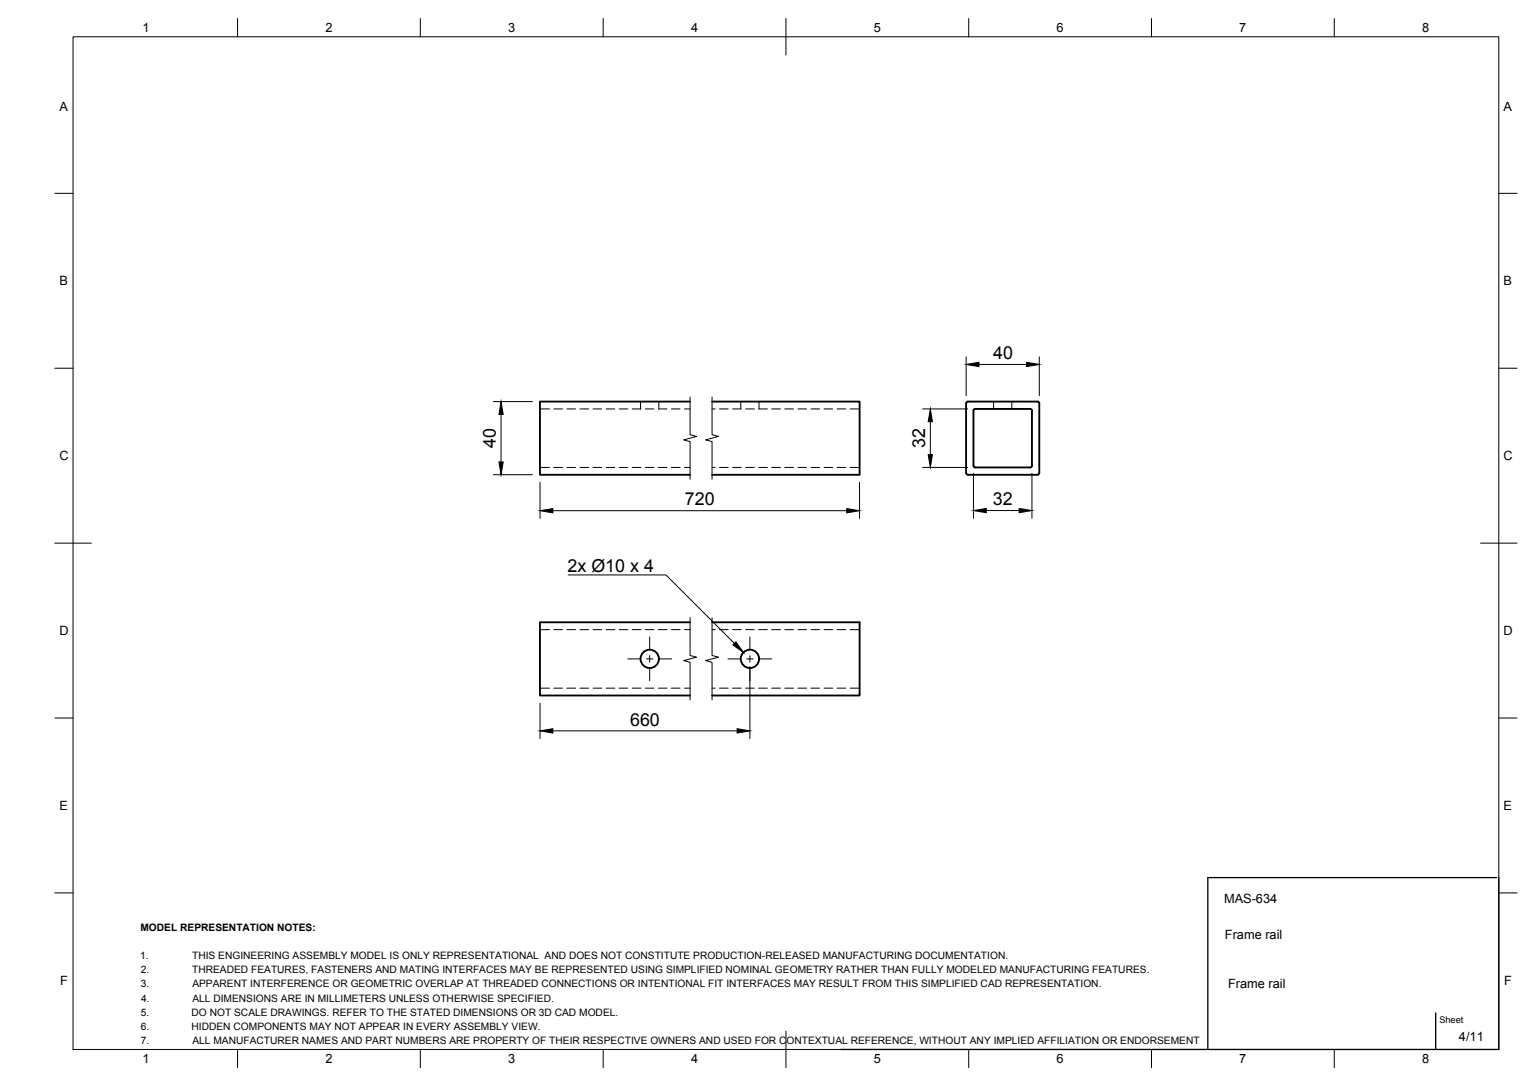
ISO-10303-21;
HEADER;
/* Generated by software containing ST-Developer
 * from STEP Tools, Inc. (www.steptools.com) 
 */

FILE_DESCRIPTION(
/* description */ ('Independent AHU equipment rack. Nominal800x600 frame on1000long40squa
re aluminum posts; two removable notched shelves; welded perimeter/cro
ss rails and rear gussets; two mounting channels; four isolation pads 
and anchor-ready feet. Imported native extrusion library retained and 
cut-length parameters customized per family. Shelf hardware uses model
ed M6 rivet nuts and screws. Weld design, floor anchors and load ratin
g require engineering selection.'),
/* implementation_level */ '2;1');

FILE_NAME(
/* name */ 'Frame rail.step',
/* time_stamp */ '2026-11-07T19:04:45-08:00',
/* author */ (''),
/* organization */ (''),
/* preprocessor_version */ 'ST-DEVELOPER v20.2',
/* originating_system */ 'Autodesk Translation Framework v15.17.0.0',
/* authorisation */ '');

FILE_SCHEMA (('AUTOMOTIVE_DESIGN { 1 0 10303 214 3 1 1 }'));
ENDSEC;

DATA;
#10=MECHANICAL_DESIGN_GEOMETRIC_PRESENTATION_REPRESENTATION('',(#336),#9777);
#314=SHAPE_REPRESENTATION_RELATIONSHIP('SRR','None',#9858,#325);
#325=ADVANCED_BREP_SHAPE_REPRESENTATION('',(#347),#9767);
#336=STYLED_ITEM('',(#9922),#347);
#347=MANIFOLD_SOLID_BREP('Aluminum square hollow profile',#3841);
#359=FACE_BOUND('',#725,.T.);
#360=FACE_BOUND('',#732,.T.);
#361=FACE_BOUND('',#733,.T.);
#362=FACE_BOUND('',#741,.T.);
#363=FACE_BOUND('',#742,.T.);
#364=FACE_BOUND('',#745,.T.);
#420=PLANE('',#4019);
#421=PLANE('',#4020);
#422=PLANE('',#4030);
#423=PLANE('',#4037);
#424=PLANE('',#4040);
#425=PLANE('',#4043);
#426=PLANE('',#4046);
#427=PLANE('',#4047);
#428=PLANE('',#4048);
#429=PLANE('',#4049);
#520=FACE_OUTER_BOUND('',#720,.T.);
#521=FACE_OUTER_BOUND('',#721,.T.);
#522=FACE_OUTER_BOUND('',#722,.T.);
#523=FACE_OUTER_BOUND('',#723,.T.);
#524=FACE_OUTER_BOUND('',#724,.T.);
#525=FACE_OUTER_BOUND('',#726,.T.);
#526=FACE_OUTER_BOUND('',#727,.T.);
#527=FACE_OUTER_BOUND('',#728,.T.);
#528=FACE_OUTER_BOUND('',#729,.T.);
#529=FACE_OUTER_BOUND('',#730,.T.);
#530=FACE_OUTER_BOUND('',#731,.T.);
#531=FACE_OUTER_BOUND('',#734,.T.);
#532=FACE_OUTER_BOUND('',#735,.T.);
#533=FACE_OUTER_BOUND('',#736,.T.);
#534=FACE_OUTER_BOUND('',#737,.T.);
#535=FACE_OUTER_BOUND('',#738,.T.);
#536=FACE_OUTER_BOUND('',#739,.T.);
#537=FACE_OUTER_BOUND('',#740,.T.);
#538=FACE_OUTER_BOUND('',#743,.T.);
#539=FACE_OUTER_BOUND('',#744,.T.);
#720=EDGE_LOOP('',(#2611,#2612,#2613,#2614));
#721=EDGE_LOOP('',(#2615,#2616,#2617,#2618));
#722=EDGE_LOOP('',(#2619,#2620,#2621,#2622));
#723=EDGE_LOOP('',(#2623,#2624,#2625,#2626));
#724=EDGE_LOOP('',(#2627,#2628,#2629,#2630,#2631,#2632,#2633,#2634));
#725=EDGE_LOOP('',(#2635,#2636,#2637,#2638,#2639,#2640,#2641,#2642));
#726=EDGE_LOOP('',(#2643,#2644,#2645,#2646));
#727=EDGE_LOOP('',(#2647,#2648,#2649,#2650));
#728=EDGE_LOOP('',(#2651,#2652,#2653,#2654));
#729=EDGE_LOOP('',(#2655,#2656,#2657,#2658));
#730=EDGE_LOOP('',(#2659,#2660,#2661,#2662));
#731=EDGE_LOOP('',(#2663,#2664,#2665,#2666));
#732=EDGE_LOOP('',(#2667));
#733=EDGE_LOOP('',(#2668));
#734=EDGE_LOOP('',(#2669,#2670,#2671,#2672));
#735=EDGE_LOOP('',(#2673,#2674,#2675,#2676));
#736=EDGE_LOOP('',(#2677,#2678,#2679,#2680));
#737=EDGE_LOOP('',(#2681,#2682,#2683,#2684));
#738=EDGE_LOOP('',(#2685,#2686,#2687,#2688));
#739=EDGE_LOOP('',(#2689,#2690,#2691,#2692));
#740=EDGE_LOOP('',(#2693,#2694,#2695,#2696));
#741=EDGE_LOOP('',(#2697));
#742=EDGE_LOOP('',(#2698));
#743=EDGE_LOOP('',(#2699,#2700,#2701,#2702));
#744=EDGE_LOOP('',(#2703,#2704,#2705,#2706,#2707,#2708,#2709,#2710));
#745=EDGE_LOOP('',(#2711,#2712,#2713,#2714,#2715,#2716,#2717,#2718));
#983=LINE('',#5508,#1276);
#984=LINE('',#5514,#1277);
#985=LINE('',#5521,#1278);
#986=LINE('',#5524,#1279);
#987=LINE('',#5527,#1280);
#988=LINE('',#5529,#1281);
#989=LINE('',#5530,#1282);
#990=LINE('',#5533,#1283);
#991=LINE('',#5537,#1284);
#992=LINE('',#5541,#1285);
#993=LINE('',#5545,#1286);
#994=LINE('',#5549,#1287);
#995=LINE('',#5553,#1288);
#996=LINE('',#5557,#1289);
#997=LINE('',#5561,#1290);
#998=LINE('',#5564,#1291);
#999=LINE('',#5567,#1292);
#1000=LINE('',#5568,#1293);
#1001=LINE('',#5572,#1294);
#1002=LINE('',#5575,#1295);
#1003=LINE('',#5581,#1296);
#1004=LINE('',#5582,#1297);
#1005=LINE('',#5585,#1298);
#1006=LINE('',#5586,#1299);
#1007=LINE('',#5590,#1300);
#1008=LINE('',#5593,#1301);
#1009=LINE('',#5594,#1302);
#1010=LINE('',#5598,#1303);
#1011=LINE('',#5601,#1304);
#1012=LINE('',#5602,#1305);
#1013=LINE('',#5606,#1306);
#1014=LINE('',#5608,#1307);
#1015=LINE('',#5610,#1308);
#1016=LINE('',#5612,#1309);
#1276=VECTOR('',#4462,5.);
#1277=VECTOR('',#4469,5.);
#1278=VECTOR('',#4476,10.);
#1279=VECTOR('',#4479,10.);
#1280=VECTOR('',#4482,10.);
#1281=VECTOR('',#4483,10.);
#1282=VECTOR('',#4484,10.);
#1283=VECTOR('',#4487,10.);
#1284=VECTOR('',#4490,10.);
#1285=VECTOR('',#4493,10.);
#1286=VECTOR('',#4496,10.);
#1287=VECTOR('',#4499,10.);
#1288=VECTOR('',#4502,10.);
#1289=VECTOR('',#4505,10.);
#1290=VECTOR('',#4510,10.);
#1291=VECTOR('',#4513,10.);
#1292=VECTOR('',#4516,10.);
#1293=VECTOR('',#4517,10.);
#1294=VECTOR('',#4522,10.);
#1295=VECTOR('',#4525,10.);
#1296=VECTOR('',#4532,10.);
#1297=VECTOR('',#4533,10.);
#1298=VECTOR('',#4536,10.);
#1299=VECTOR('',#4537,10.);
#1300=VECTOR('',#4542,10.);
#1301=VECTOR('',#4545,10.);
#1302=VECTOR('',#4546,10.);
#1303=VECTOR('',#4551,10.);
#1304=VECTOR('',#4554,10.);
#1305=VECTOR('',#4555,10.);
#1306=VECTOR('',#4560,10.);
#1307=VECTOR('',#4563,10.);
#1308=VECTOR('',#4566,10.);
#1309=VECTOR('',#4569,10.);
#1553=CIRCLE('',#4011,5.);
#1554=CIRCLE('',#4012,5.);
#1555=CIRCLE('',#4014,5.);
#1556=CIRCLE('',#4015,5.);
#1557=CIRCLE('',#4017,1.);
#1558=CIRCLE('',#4018,1.);
#1559=CIRCLE('',#4021,1.);
#1560=CIRCLE('',#4022,1.);
#1561=CIRCLE('',#4023,1.);
#1562=CIRCLE('',#4024,1.);
#1563=CIRCLE('',#4025,1.);
#1564=CIRCLE('',#4026,1.);
#1565=CIRCLE('',#4027,1.);
#1566=CIRCLE('',#4029,1.);
#1567=CIRCLE('',#4032,1.);
#1568=CIRCLE('',#4034,1.);
#1569=CIRCLE('',#4036,1.);
#1570=CIRCLE('',#4039,1.);
#1571=CIRCLE('',#4042,1.);
#1572=CIRCLE('',#4045,1.);
#1692=VERTEX_POINT('',#5505);
#1693=VERTEX_POINT('',#5507);
#1694=VERTEX_POINT('',#5511);
#1695=VERTEX_POINT('',#5513);
#1696=VERTEX_POINT('',#5517);
#1697=VERTEX_POINT('',#5518);
#1698=VERTEX_POINT('',#5520);
#1699=VERTEX_POINT('',#5522);
#1700=VERTEX_POINT('',#5526);
#1701=VERTEX_POINT('',#5528);
#1702=VERTEX_POINT('',#5532);
#1703=VERTEX_POINT('',#5534);
#1704=VERTEX_POINT('',#5536);
#1705=VERTEX_POINT('',#5538);
#1706=VERTEX_POINT('',#5540);
#1707=VERTEX_POINT('',#5543);
#1708=VERTEX_POINT('',#5544);
#1709=VERTEX_POINT('',#5546);
#1710=VERTEX_POINT('',#5548);
#1711=VERTEX_POINT('',#5550);
#1712=VERTEX_POINT('',#5552);
#1713=VERTEX_POINT('',#5554);
#1714=VERTEX_POINT('',#5556);
#1715=VERTEX_POINT('',#5560);
#1716=VERTEX_POINT('',#5562);
#1717=VERTEX_POINT('',#5566);
#1718=VERTEX_POINT('',#5570);
#1719=VERTEX_POINT('',#5574);
#1720=VERTEX_POINT('',#5578);
#1721=VERTEX_POINT('',#5579);
#1722=VERTEX_POINT('',#5584);
#1723=VERTEX_POINT('',#5588);
#1724=VERTEX_POINT('',#5592);
#1725=VERTEX_POINT('',#5596);
#1726=VERTEX_POINT('',#5600);
#1727=VERTEX_POINT('',#5604);
#2050=EDGE_CURVE('',#1692,#1692,#1553,.T.);
#2051=EDGE_CURVE('',#1692,#1693,#983,.T.);
#2052=EDGE_CURVE('',#1693,#1693,#1554,.T.);
#2053=EDGE_CURVE('',#1694,#1694,#1555,.T.);
#2054=EDGE_CURVE('',#1694,#1695,#984,.T.);
#2055=EDGE_CURVE('',#1695,#1695,#1556,.T.);
#2056=EDGE_CURVE('',#1696,#1697,#1557,.T.);
#2057=EDGE_CURVE('',#1697,#1698,#985,.T.);
#2058=EDGE_CURVE('',#1698,#1699,#1558,.T.);
#2059=EDGE_CURVE('',#1699,#1696,#986,.T.);
#2060=EDGE_CURVE('',#1700,#1697,#987,.T.);
#2061=EDGE_CURVE('',#1701,#1700,#988,.T.);
#2062=EDGE_CURVE('',#1701,#1698,#989,.T.);
#2063=EDGE_CURVE('',#1696,#1702,#990,.T.);
#2064=EDGE_CURVE('',#1703,#1702,#1559,.T.);
#2065=EDGE_CURVE('',#1703,#1704,#991,.T.);
#2066=EDGE_CURVE('',#1705,#1704,#1560,.T.);
#2067=EDGE_CURVE('',#1705,#1706,#992,.T.);
#2068=EDGE_CURVE('',#1700,#1706,#1561,.T.);
#2069=EDGE_CURVE('',#1707,#1708,#993,.T.);
#2070=EDGE_CURVE('',#1709,#1708,#1562,.T.);
#2071=EDGE_CURVE('',#1709,#1710,#994,.T.);
#2072=EDGE_CURVE('',#1711,#1710,#1563,.T.);
#2073=EDGE_CURVE('',#1711,#1712,#995,.T.);
#2074=EDGE_CURVE('',#1713,#1712,#1564,.T.);
#2075=EDGE_CURVE('',#1713,#1714,#996,.T.);
#2076=EDGE_CURVE('',#1707,#1714,#1565,.T.);
#2077=EDGE_CURVE('',#1702,#1715,#997,.T.);
#2078=EDGE_CURVE('',#1715,#1716,#1566,.T.);
#2079=EDGE_CURVE('',#1716,#1703,#998,.T.);
#2080=EDGE_CURVE('',#1716,#1717,#999,.T.);
#2081=EDGE_CURVE('',#1704,#1717,#1000,.T.);
#2082=EDGE_CURVE('',#1717,#1718,#1567,.T.);
#2083=EDGE_CURVE('',#1718,#1705,#1001,.T.);
#2084=EDGE_CURVE('',#1706,#1719,#1002,.T.);
#2085=EDGE_CURVE('',#1719,#1701,#1568,.T.);
#2086=EDGE_CURVE('',#1720,#1721,#1569,.T.);
#2087=EDGE_CURVE('',#1721,#1709,#1003,.T.);
#2088=EDGE_CURVE('',#1708,#1720,#1004,.T.);
#2089=EDGE_CURVE('',#1721,#1722,#1005,.T.);
#2090=EDGE_CURVE('',#1710,#1722,#1006,.T.);
#2091=EDGE_CURVE('',#1722,#1723,#1570,.T.);
#2092=EDGE_CURVE('',#1723,#1711,#1007,.T.);
#2093=EDGE_CURVE('',#1723,#1724,#1008,.T.);
#2094=EDGE_CURVE('',#1712,#1724,#1009,.T.);
#2095=EDGE_CURVE('',#1724,#1725,#1571,.T.);
#2096=EDGE_CURVE('',#1725,#1713,#1010,.T.);
#2097=EDGE_CURVE('',#1725,#1726,#1011,.T.);
#2098=EDGE_CURVE('',#1714,#1726,#1012,.T.);
#2099=EDGE_CURVE('',#1726,#1727,#1572,.T.);
#2100=EDGE_CURVE('',#1727,#1707,#1013,.T.);
#2101=EDGE_CURVE('',#1727,#1720,#1014,.T.);
#2102=EDGE_CURVE('',#1718,#1719,#1015,.T.);
#2103=EDGE_CURVE('',#1699,#1715,#1016,.T.);
#2611=ORIENTED_EDGE('',*,*,#2050,.F.);
#2612=ORIENTED_EDGE('',*,*,#2051,.T.);
#2613=ORIENTED_EDGE('',*,*,#2052,.F.);
#2614=ORIENTED_EDGE('',*,*,#2051,.F.);
#2615=ORIENTED_EDGE('',*,*,#2053,.F.);
#2616=ORIENTED_EDGE('',*,*,#2054,.T.);
#2617=ORIENTED_EDGE('',*,*,#2055,.F.);
#2618=ORIENTED_EDGE('',*,*,#2054,.F.);
#2619=ORIENTED_EDGE('',*,*,#2056,.T.);
#2620=ORIENTED_EDGE('',*,*,#2057,.T.);
#2621=ORIENTED_EDGE('',*,*,#2058,.T.);
#2622=ORIENTED_EDGE('',*,*,#2059,.T.);
#2623=ORIENTED_EDGE('',*,*,#2057,.F.);
#2624=ORIENTED_EDGE('',*,*,#2060,.F.);
#2625=ORIENTED_EDGE('',*,*,#2061,.F.);
#2626=ORIENTED_EDGE('',*,*,#2062,.T.);
#2627=ORIENTED_EDGE('',*,*,#2056,.F.);
#2628=ORIENTED_EDGE('',*,*,#2063,.T.);
#2629=ORIENTED_EDGE('',*,*,#2064,.F.);
#2630=ORIENTED_EDGE('',*,*,#2065,.T.);
#2631=ORIENTED_EDGE('',*,*,#2066,.F.);
#2632=ORIENTED_EDGE('',*,*,#2067,.T.);
#2633=ORIENTED_EDGE('',*,*,#2068,.F.);
#2634=ORIENTED_EDGE('',*,*,#2060,.T.);
#2635=ORIENTED_EDGE('',*,*,#2069,.T.);
#2636=ORIENTED_EDGE('',*,*,#2070,.F.);
#2637=ORIENTED_EDGE('',*,*,#2071,.T.);
#2638=ORIENTED_EDGE('',*,*,#2072,.F.);
#2639=ORIENTED_EDGE('',*,*,#2073,.T.);
#2640=ORIENTED_EDGE('',*,*,#2074,.F.);
#2641=ORIENTED_EDGE('',*,*,#2075,.T.);
#2642=ORIENTED_EDGE('',*,*,#2076,.F.);
#2643=ORIENTED_EDGE('',*,*,#2064,.T.);
#2644=ORIENTED_EDGE('',*,*,#2077,.T.);
#2645=ORIENTED_EDGE('',*,*,#2078,.T.);
#2646=ORIENTED_EDGE('',*,*,#2079,.T.);
#2647=ORIENTED_EDGE('',*,*,#2079,.F.);
#2648=ORIENTED_EDGE('',*,*,#2080,.T.);
#2649=ORIENTED_EDGE('',*,*,#2081,.F.);
#2650=ORIENTED_EDGE('',*,*,#2065,.F.);
#2651=ORIENTED_EDGE('',*,*,#2066,.T.);
#2652=ORIENTED_EDGE('',*,*,#2081,.T.);
#2653=ORIENTED_EDGE('',*,*,#2082,.T.);
#2654=ORIENTED_EDGE('',*,*,#2083,.T.);
#2655=ORIENTED_EDGE('',*,*,#2068,.T.);
#2656=ORIENTED_EDGE('',*,*,#2084,.T.);
#2657=ORIENTED_EDGE('',*,*,#2085,.T.);
#2658=ORIENTED_EDGE('',*,*,#2061,.T.);
#2659=ORIENTED_EDGE('',*,*,#2086,.T.);
#2660=ORIENTED_EDGE('',*,*,#2087,.T.);
#2661=ORIENTED_EDGE('',*,*,#2070,.T.);
#2662=ORIENTED_EDGE('',*,*,#2088,.T.);
#2663=ORIENTED_EDGE('',*,*,#2087,.F.);
#2664=ORIENTED_EDGE('',*,*,#2089,.T.);
#2665=ORIENTED_EDGE('',*,*,#2090,.F.);
#2666=ORIENTED_EDGE('',*,*,#2071,.F.);
#2667=ORIENTED_EDGE('',*,*,#2052,.T.);
#2668=ORIENTED_EDGE('',*,*,#2055,.T.);
#2669=ORIENTED_EDGE('',*,*,#2091,.T.);
#2670=ORIENTED_EDGE('',*,*,#2092,.T.);
#2671=ORIENTED_EDGE('',*,*,#2072,.T.);
#2672=ORIENTED_EDGE('',*,*,#2090,.T.);
#2673=ORIENTED_EDGE('',*,*,#2092,.F.);
#2674=ORIENTED_EDGE('',*,*,#2093,.T.);
#2675=ORIENTED_EDGE('',*,*,#2094,.F.);
#2676=ORIENTED_EDGE('',*,*,#2073,.F.);
#2677=ORIENTED_EDGE('',*,*,#2095,.T.);
#2678=ORIENTED_EDGE('',*,*,#2096,.T.);
#2679=ORIENTED_EDGE('',*,*,#2074,.T.);
#2680=ORIENTED_EDGE('',*,*,#2094,.T.);
#2681=ORIENTED_EDGE('',*,*,#2096,.F.);
#2682=ORIENTED_EDGE('',*,*,#2097,.T.);
#2683=ORIENTED_EDGE('',*,*,#2098,.F.);
#2684=ORIENTED_EDGE('',*,*,#2075,.F.);
#2685=ORIENTED_EDGE('',*,*,#2099,.T.);
#2686=ORIENTED_EDGE('',*,*,#2100,.T.);
#2687=ORIENTED_EDGE('',*,*,#2076,.T.);
#2688=ORIENTED_EDGE('',*,*,#2098,.T.);
#2689=ORIENTED_EDGE('',*,*,#2088,.F.);
#2690=ORIENTED_EDGE('',*,*,#2069,.F.);
#2691=ORIENTED_EDGE('',*,*,#2100,.F.);
#2692=ORIENTED_EDGE('',*,*,#2101,.T.);
#2693=ORIENTED_EDGE('',*,*,#2083,.F.);
#2694=ORIENTED_EDGE('',*,*,#2102,.T.);
#2695=ORIENTED_EDGE('',*,*,#2084,.F.);
#2696=ORIENTED_EDGE('',*,*,#2067,.F.);
#2697=ORIENTED_EDGE('',*,*,#2050,.T.);
#2698=ORIENTED_EDGE('',*,*,#2053,.T.);
#2699=ORIENTED_EDGE('',*,*,#2059,.F.);
#2700=ORIENTED_EDGE('',*,*,#2103,.T.);
#2701=ORIENTED_EDGE('',*,*,#2077,.F.);
#2702=ORIENTED_EDGE('',*,*,#2063,.F.);
#2703=ORIENTED_EDGE('',*,*,#2058,.F.);
#2704=ORIENTED_EDGE('',*,*,#2062,.F.);
#2705=ORIENTED_EDGE('',*,*,#2085,.F.);
#2706=ORIENTED_EDGE('',*,*,#2102,.F.);
#2707=ORIENTED_EDGE('',*,*,#2082,.F.);
#2708=ORIENTED_EDGE('',*,*,#2080,.F.);
#2709=ORIENTED_EDGE('',*,*,#2078,.F.);
#2710=ORIENTED_EDGE('',*,*,#2103,.F.);
#2711=ORIENTED_EDGE('',*,*,#2099,.F.);
#2712=ORIENTED_EDGE('',*,*,#2097,.F.);
#2713=ORIENTED_EDGE('',*,*,#2095,.F.);
#2714=ORIENTED_EDGE('',*,*,#2093,.F.);
#2715=ORIENTED_EDGE('',*,*,#2091,.F.);
#2716=ORIENTED_EDGE('',*,*,#2089,.F.);
#2717=ORIENTED_EDGE('',*,*,#2086,.F.);
#2718=ORIENTED_EDGE('',*,*,#2101,.F.);
#3549=CYLINDRICAL_SURFACE('',#4010,5.);
#3550=CYLINDRICAL_SURFACE('',#4013,5.);
#3551=CYLINDRICAL_SURFACE('',#4016,1.);
#3552=CYLINDRICAL_SURFACE('',#4028,1.);
#3553=CYLINDRICAL_SURFACE('',#4031,1.);
#3554=CYLINDRICAL_SURFACE('',#4033,1.);
#3555=CYLINDRICAL_SURFACE('',#4035,1.);
#3556=CYLINDRICAL_SURFACE('',#4038,1.);
#3557=CYLINDRICAL_SURFACE('',#4041,1.);
#3558=CYLINDRICAL_SURFACE('',#4044,1.);
#3660=ADVANCED_FACE('',(#520),#3549,.F.);
#3661=ADVANCED_FACE('',(#521),#3550,.F.);
#3662=ADVANCED_FACE('',(#522),#3551,.T.);
#3663=ADVANCED_FACE('',(#523),#420,.T.);
#3664=ADVANCED_FACE('',(#524,#359),#421,.T.);
#3665=ADVANCED_FACE('',(#525),#3552,.T.);
#3666=ADVANCED_FACE('',(#526),#422,.T.);
#3667=ADVANCED_FACE('',(#527),#3553,.T.);
#3668=ADVANCED_FACE('',(#528),#3554,.T.);
#3669=ADVANCED_FACE('',(#529),#3555,.F.);
#3670=ADVANCED_FACE('',(#530,#360,#361),#423,.T.);
#3671=ADVANCED_FACE('',(#531),#3556,.F.);
#3672=ADVANCED_FACE('',(#532),#424,.T.);
#3673=ADVANCED_FACE('',(#533),#3557,.F.);
#3674=ADVANCED_FACE('',(#534),#425,.T.);
#3675=ADVANCED_FACE('',(#535),#3558,.F.);
#3676=ADVANCED_FACE('',(#536),#426,.T.);
#3677=ADVANCED_FACE('',(#537,#362,#363),#427,.T.);
#3678=ADVANCED_FACE('',(#538),#428,.T.);
#3679=ADVANCED_FACE('',(#539,#364),#429,.F.);
#3841=CLOSED_SHELL('',(#3660,#3661,#3662,#3663,#3664,#3665,#3666,#3667,
#3668,#3669,#3670,#3671,#3672,#3673,#3674,#3675,#3676,#3677,#3678,#3679));
#4009=AXIS2_PLACEMENT_3D('',#5503,#4456,#4457);
#4010=AXIS2_PLACEMENT_3D('',#5504,#4458,#4459);
#4011=AXIS2_PLACEMENT_3D('',#5506,#4460,#4461);
#4012=AXIS2_PLACEMENT_3D('',#5509,#4463,#4464);
#4013=AXIS2_PLACEMENT_3D('',#5510,#4465,#4466);
#4014=AXIS2_PLACEMENT_3D('',#5512,#4467,#4468);
#4015=AXIS2_PLACEMENT_3D('',#5515,#4470,#4471);
#4016=AXIS2_PLACEMENT_3D('',#5516,#4472,#4473);
#4017=AXIS2_PLACEMENT_3D('',#5519,#4474,#4475);
#4018=AXIS2_PLACEMENT_3D('',#5523,#4477,#4478);
#4019=AXIS2_PLACEMENT_3D('',#5525,#4480,#4481);
#4020=AXIS2_PLACEMENT_3D('',#5531,#4485,#4486);
#4021=AXIS2_PLACEMENT_3D('',#5535,#4488,#4489);
#4022=AXIS2_PLACEMENT_3D('',#5539,#4491,#4492);
#4023=AXIS2_PLACEMENT_3D('',#5542,#4494,#4495);
#4024=AXIS2_PLACEMENT_3D('',#5547,#4497,#4498);
#4025=AXIS2_PLACEMENT_3D('',#5551,#4500,#4501);
#4026=AXIS2_PLACEMENT_3D('',#5555,#4503,#4504);
#4027=AXIS2_PLACEMENT_3D('',#5558,#4506,#4507);
#4028=AXIS2_PLACEMENT_3D('',#5559,#4508,#4509);
#4029=AXIS2_PLACEMENT_3D('',#5563,#4511,#4512);
#4030=AXIS2_PLACEMENT_3D('',#5565,#4514,#4515);
#4031=AXIS2_PLACEMENT_3D('',#5569,#4518,#4519);
#4032=AXIS2_PLACEMENT_3D('',#5571,#4520,#4521);
#4033=AXIS2_PLACEMENT_3D('',#5573,#4523,#4524);
#4034=AXIS2_PLACEMENT_3D('',#5576,#4526,#4527);
#4035=AXIS2_PLACEMENT_3D('',#5577,#4528,#4529);
#4036=AXIS2_PLACEMENT_3D('',#5580,#4530,#4531);
#4037=AXIS2_PLACEMENT_3D('',#5583,#4534,#4535);
#4038=AXIS2_PLACEMENT_3D('',#5587,#4538,#4539);
#4039=AXIS2_PLACEMENT_3D('',#5589,#4540,#4541);
#4040=AXIS2_PLACEMENT_3D('',#5591,#4543,#4544);
#4041=AXIS2_PLACEMENT_3D('',#5595,#4547,#4548);
#4042=AXIS2_PLACEMENT_3D('',#5597,#4549,#4550);
#4043=AXIS2_PLACEMENT_3D('',#5599,#4552,#4553);
#4044=AXIS2_PLACEMENT_3D('',#5603,#4556,#4557);
#4045=AXIS2_PLACEMENT_3D('',#5605,#4558,#4559);
#4046=AXIS2_PLACEMENT_3D('',#5607,#4561,#4562);
#4047=AXIS2_PLACEMENT_3D('',#5609,#4564,#4565);
#4048=AXIS2_PLACEMENT_3D('',#5611,#4567,#4568);
#4049=AXIS2_PLACEMENT_3D('',#5613,#4570,#4571);
#4456=DIRECTION('axis',(0.,0.,1.));
#4457=DIRECTION('refdir',(1.,0.,0.));
#4458=DIRECTION('center_axis',(0.,-1.,0.));
#4459=DIRECTION('ref_axis',(0.,0.,1.));
#4460=DIRECTION('center_axis',(0.,-1.,0.));
#4461=DIRECTION('ref_axis',(0.,0.,1.));
#4462=DIRECTION('',(0.,-1.,0.));
#4463=DIRECTION('center_axis',(0.,1.,0.));
#4464=DIRECTION('ref_axis',(0.,0.,1.));
#4465=DIRECTION('center_axis',(0.,-1.,0.));
#4466=DIRECTION('ref_axis',(0.,0.,1.));
#4467=DIRECTION('center_axis',(0.,-1.,0.));
#4468=DIRECTION('ref_axis',(0.,0.,1.));
#4469=DIRECTION('',(0.,-1.,0.));
#4470=DIRECTION('center_axis',(0.,1.,0.));
#4471=DIRECTION('ref_axis',(0.,0.,1.));
#4472=DIRECTION('center_axis',(0.,0.,1.));
#4473=DIRECTION('ref_axis',(-0.707106781186548,-0.707106781186548,0.));
#4474=DIRECTION('center_axis',(0.,0.,-1.));
#4475=DIRECTION('ref_axis',(-0.707106781186548,-0.707106781186548,0.));
#4476=DIRECTION('',(0.,0.,-1.));
#4477=DIRECTION('center_axis',(0.,0.,1.));
#4478=DIRECTION('ref_axis',(-0.707106781186548,-0.707106781186548,0.));
#4479=DIRECTION('',(0.,0.,1.));
#4480=DIRECTION('center_axis',(-1.,0.,0.));
#4481=DIRECTION('ref_axis',(0.,-1.,0.));
#4482=DIRECTION('',(0.,-1.,0.));
#4483=DIRECTION('',(0.,0.,1.));
#4484=DIRECTION('',(0.,-1.,0.));
#4485=DIRECTION('center_axis',(0.,0.,1.));
#4486=DIRECTION('ref_axis',(1.,0.,0.));
#4487=DIRECTION('',(1.,0.,0.));
#4488=DIRECTION('center_axis',(0.,0.,-1.));
#4489=DIRECTION('ref_axis',(0.707106781186548,-0.707106781186548,0.));
#4490=DIRECTION('',(0.,1.,0.));
#4491=DIRECTION('center_axis',(0.,0.,-1.));
#4492=DIRECTION('ref_axis',(0.707106781186548,0.707106781186548,0.));
#4493=DIRECTION('',(-1.,0.,0.));
#4494=DIRECTION('center_axis',(0.,0.,-1.));
#4495=DIRECTION('ref_axis',(-0.707106781186548,0.707106781186548,0.));
#4496=DIRECTION('',(0.,1.,0.));
#4497=DIRECTION('center_axis',(0.,0.,1.));
#4498=DIRECTION('ref_axis',(-0.707106781186548,0.707106781186548,0.));
#4499=DIRECTION('',(1.,0.,0.));
#4500=DIRECTION('center_axis',(0.,0.,1.));
#4501=DIRECTION('ref_axis',(0.707106781186548,0.707106781186548,0.));
#4502=DIRECTION('',(0.,-1.,0.));
#4503=DIRECTION('center_axis',(0.,0.,1.));
#4504=DIRECTION('ref_axis',(0.707106781186548,-0.707106781186548,0.));
#4505=DIRECTION('',(-1.,0.,0.));
#4506=DIRECTION('center_axis',(0.,0.,1.));
#4507=DIRECTION('ref_axis',(-0.707106781186548,-0.707106781186548,0.));
#4508=DIRECTION('center_axis',(0.,0.,1.));
#4509=DIRECTION('ref_axis',(0.707106781186548,-0.707106781186548,0.));
#4510=DIRECTION('',(0.,0.,-1.));
#4511=DIRECTION('center_axis',(0.,0.,1.));
#4512=DIRECTION('ref_axis',(0.707106781186548,-0.707106781186548,0.));
#4513=DIRECTION('',(0.,0.,1.));
#4514=DIRECTION('center_axis',(1.,0.,0.));
#4515=DIRECTION('ref_axis',(0.,1.,0.));
#4516=DIRECTION('',(0.,1.,0.));
#4517=DIRECTION('',(0.,0.,-1.));
#4518=DIRECTION('center_axis',(0.,0.,1.));
#4519=DIRECTION('ref_axis',(0.707106781186548,0.707106781186548,0.));
#4520=DIRECTION('center_axis',(0.,0.,1.));
#4521=DIRECTION('ref_axis',(0.707106781186548,0.707106781186548,0.));
#4522=DIRECTION('',(0.,0.,1.));
#4523=DIRECTION('center_axis',(0.,0.,1.));
#4524=DIRECTION('ref_axis',(-0.707106781186548,0.707106781186548,0.));
#4525=DIRECTION('',(0.,0.,-1.));
#4526=DIRECTION('center_axis',(0.,0.,1.));
#4527=DIRECTION('ref_axis',(-0.707106781186548,0.707106781186548,0.));
#4528=DIRECTION('center_axis',(0.,0.,1.));
#4529=DIRECTION('ref_axis',(-0.707106781186548,0.707106781186548,0.));
#4530=DIRECTION('center_axis',(0.,0.,-1.));
#4531=DIRECTION('ref_axis',(-0.707106781186548,0.707106781186548,0.));
#4532=DIRECTION('',(0.,0.,1.));
#4533=DIRECTION('',(0.,0.,-1.));
#4534=DIRECTION('center_axis',(0.,-1.,0.));
#4535=DIRECTION('ref_axis',(1.,0.,0.));
#4536=DIRECTION('',(1.,0.,0.));
#4537=DIRECTION('',(0.,0.,-1.));
#4538=DIRECTION('center_axis',(0.,0.,1.));
#4539=DIRECTION('ref_axis',(0.707106781186548,0.707106781186548,0.));
#4540=DIRECTION('center_axis',(0.,0.,-1.));
#4541=DIRECTION('ref_axis',(0.707106781186548,0.707106781186548,0.));
#4542=DIRECTION('',(0.,0.,1.));
#4543=DIRECTION('center_axis',(-1.,0.,0.));
#4544=DIRECTION('ref_axis',(0.,-1.,0.));
#4545=DIRECTION('',(0.,-1.,0.));
#4546=DIRECTION('',(0.,0.,-1.));
#4547=DIRECTION('center_axis',(0.,0.,1.));
#4548=DIRECTION('ref_axis',(0.707106781186548,-0.707106781186548,0.));
#4549=DIRECTION('center_axis',(0.,0.,-1.));
#4550=DIRECTION('ref_axis',(0.707106781186548,-0.707106781186548,0.));
#4551=DIRECTION('',(0.,0.,1.));
#4552=DIRECTION('center_axis',(0.,1.,0.));
#4553=DIRECTION('ref_axis',(-1.,0.,0.));
#4554=DIRECTION('',(-1.,0.,0.));
#4555=DIRECTION('',(0.,0.,-1.));
#4556=DIRECTION('center_axis',(0.,0.,1.));
#4557=DIRECTION('ref_axis',(-0.707106781186548,-0.707106781186548,0.));
#4558=DIRECTION('center_axis',(0.,0.,-1.));
#4559=DIRECTION('ref_axis',(-0.707106781186548,-0.707106781186548,0.));
#4560=DIRECTION('',(0.,0.,1.));
#4561=DIRECTION('center_axis',(1.,0.,0.));
#4562=DIRECTION('ref_axis',(0.,1.,0.));
#4563=DIRECTION('',(0.,1.,0.));
#4564=DIRECTION('center_axis',(0.,1.,0.));
#4565=DIRECTION('ref_axis',(-1.,0.,0.));
#4566=DIRECTION('',(-1.,0.,0.));
#4567=DIRECTION('center_axis',(0.,-1.,0.));
#4568=DIRECTION('ref_axis',(1.,0.,0.));
#4569=DIRECTION('',(1.,0.,0.));
#4570=DIRECTION('center_axis',(0.,0.,1.));
#4571=DIRECTION('ref_axis',(1.,0.,0.));
#5503=CARTESIAN_POINT('',(0.,0.,0.));
#5504=CARTESIAN_POINT('Origin',(0.,18.,60.));
#5505=CARTESIAN_POINT('',(6.12323399573677E-16,20.,55.));
#5506=CARTESIAN_POINT('Origin',(0.,20.,60.));
#5507=CARTESIAN_POINT('',(6.12323399573677E-16,16.,55.));
#5508=CARTESIAN_POINT('',(6.12323399573677E-16,18.,55.));
#5509=CARTESIAN_POINT('Origin',(0.,16.,60.));
#5510=CARTESIAN_POINT('Origin',(0.,18.,660.));
#5511=CARTESIAN_POINT('',(6.12323399573677E-16,20.,655.));
#5512=CARTESIAN_POINT('Origin',(0.,20.,660.));
#5513=CARTESIAN_POINT('',(6.12323399573677E-16,16.,655.));
#5514=CARTESIAN_POINT('',(6.12323399573677E-16,18.,655.));
#5515=CARTESIAN_POINT('Origin',(0.,16.,660.));
#5516=CARTESIAN_POINT('Origin',(-19.,-19.,0.));
#5517=CARTESIAN_POINT('',(-19.,-20.,720.));
#5518=CARTESIAN_POINT('',(-20.,-19.,720.));
#5519=CARTESIAN_POINT('Origin',(-19.,-19.,720.));
#5520=CARTESIAN_POINT('',(-20.,-19.,0.));
#5521=CARTESIAN_POINT('',(-20.,-19.,0.));
#5522=CARTESIAN_POINT('',(-19.,-20.,0.));
#5523=CARTESIAN_POINT('Origin',(-19.,-19.,0.));
#5524=CARTESIAN_POINT('',(-19.,-20.,0.));
#5525=CARTESIAN_POINT('Origin',(-20.,20.,0.));
#5526=CARTESIAN_POINT('',(-20.,19.,720.));
#5527=CARTESIAN_POINT('',(-20.,20.,720.));
#5528=CARTESIAN_POINT('',(-20.,19.,0.));
#5529=CARTESIAN_POINT('',(-20.,19.,0.));
#5530=CARTESIAN_POINT('',(-20.,20.,0.));
#5531=CARTESIAN_POINT('Origin',(0.,0.,720.));
#5532=CARTESIAN_POINT('',(19.,-20.,720.));
#5533=CARTESIAN_POINT('',(-20.,-20.,720.));
#5534=CARTESIAN_POINT('',(20.,-19.,720.));
#5535=CARTESIAN_POINT('Origin',(19.,-19.,720.));
#5536=CARTESIAN_POINT('',(20.,19.,720.));
#5537=CARTESIAN_POINT('',(20.,-20.,720.));
#5538=CARTESIAN_POINT('',(19.,20.,720.));
#5539=CARTESIAN_POINT('Origin',(19.,19.,720.));
#5540=CARTESIAN_POINT('',(-19.,20.,720.));
#5541=CARTESIAN_POINT('',(20.,20.,720.));
#5542=CARTESIAN_POINT('Origin',(-19.,19.,720.));
#5543=CARTESIAN_POINT('',(-16.,-15.,720.));
#5544=CARTESIAN_POINT('',(-16.,15.,720.));
#5545=CARTESIAN_POINT('',(-16.,16.,720.));
#5546=CARTESIAN_POINT('',(-15.,16.,720.));
#5547=CARTESIAN_POINT('Origin',(-15.,15.,720.));
#5548=CARTESIAN_POINT('',(15.,16.,720.));
#5549=CARTESIAN_POINT('',(16.,16.,720.));
#5550=CARTESIAN_POINT('',(16.,15.,720.));
#5551=CARTESIAN_POINT('Origin',(15.,15.,720.));
#5552=CARTESIAN_POINT('',(16.,-15.,720.));
#5553=CARTESIAN_POINT('',(16.,-16.,720.));
#5554=CARTESIAN_POINT('',(15.,-16.,720.));
#5555=CARTESIAN_POINT('Origin',(15.,-15.,720.));
#5556=CARTESIAN_POINT('',(-15.,-16.,720.));
#5557=CARTESIAN_POINT('',(-16.,-16.,720.));
#5558=CARTESIAN_POINT('Origin',(-15.,-15.,720.));
#5559=CARTESIAN_POINT('Origin',(19.,-19.,0.));
#5560=CARTESIAN_POINT('',(19.,-20.,0.));
#5561=CARTESIAN_POINT('',(19.,-20.,0.));
#5562=CARTESIAN_POINT('',(20.,-19.,0.));
#5563=CARTESIAN_POINT('Origin',(19.,-19.,0.));
#5564=CARTESIAN_POINT('',(20.,-19.,0.));
#5565=CARTESIAN_POINT('Origin',(20.,-20.,0.));
#5566=CARTESIAN_POINT('',(20.,19.,0.));
#5567=CARTESIAN_POINT('',(20.,-20.,0.));
#5568=CARTESIAN_POINT('',(20.,19.,0.));
#5569=CARTESIAN_POINT('Origin',(19.,19.,0.));
#5570=CARTESIAN_POINT('',(19.,20.,0.));
#5571=CARTESIAN_POINT('Origin',(19.,19.,0.));
#5572=CARTESIAN_POINT('',(19.,20.,0.));
#5573=CARTESIAN_POINT('Origin',(-19.,19.,0.));
#5574=CARTESIAN_POINT('',(-19.,20.,0.));
#5575=CARTESIAN_POINT('',(-19.,20.,0.));
#5576=CARTESIAN_POINT('Origin',(-19.,19.,0.));
#5577=CARTESIAN_POINT('Origin',(-15.,15.,0.));
#5578=CARTESIAN_POINT('',(-16.,15.,0.));
#5579=CARTESIAN_POINT('',(-15.,16.,0.));
#5580=CARTESIAN_POINT('Origin',(-15.,15.,0.));
#5581=CARTESIAN_POINT('',(-15.,16.,0.));
#5582=CARTESIAN_POINT('',(-16.,15.,0.));
#5583=CARTESIAN_POINT('Origin',(-16.,16.,0.));
#5584=CARTESIAN_POINT('',(15.,16.,0.));
#5585=CARTESIAN_POINT('',(16.,16.,0.));
#5586=CARTESIAN_POINT('',(15.,16.,0.));
#5587=CARTESIAN_POINT('Origin',(15.,15.,0.));
#5588=CARTESIAN_POINT('',(16.,15.,0.));
#5589=CARTESIAN_POINT('Origin',(15.,15.,0.));
#5590=CARTESIAN_POINT('',(16.,15.,0.));
#5591=CARTESIAN_POINT('Origin',(16.,16.,0.));
#5592=CARTESIAN_POINT('',(16.,-15.,0.));
#5593=CARTESIAN_POINT('',(16.,-16.,0.));
#5594=CARTESIAN_POINT('',(16.,-15.,0.));
#5595=CARTESIAN_POINT('Origin',(15.,-15.,0.));
#5596=CARTESIAN_POINT('',(15.,-16.,0.));
#5597=CARTESIAN_POINT('Origin',(15.,-15.,0.));
#5598=CARTESIAN_POINT('',(15.,-16.,0.));
#5599=CARTESIAN_POINT('Origin',(16.,-16.,0.));
#5600=CARTESIAN_POINT('',(-15.,-16.,0.));
#5601=CARTESIAN_POINT('',(-16.,-16.,0.));
#5602=CARTESIAN_POINT('',(-15.,-16.,0.));
#5603=CARTESIAN_POINT('Origin',(-15.,-15.,0.));
#5604=CARTESIAN_POINT('',(-16.,-15.,0.));
#5605=CARTESIAN_POINT('Origin',(-15.,-15.,0.));
#5606=CARTESIAN_POINT('',(-16.,-15.,0.));
#5607=CARTESIAN_POINT('Origin',(-16.,-16.,0.));
#5608=CARTESIAN_POINT('',(-16.,16.,0.));
#5609=CARTESIAN_POINT('Origin',(20.,20.,0.));
#5610=CARTESIAN_POINT('',(20.,20.,0.));
#5611=CARTESIAN_POINT('Origin',(-20.,-20.,0.));
#5612=CARTESIAN_POINT('',(-20.,-20.,0.));
#5613=CARTESIAN_POINT('Origin',(0.,0.,0.));
#9754=UNCERTAINTY_MEASURE_WITH_UNIT(LENGTH_MEASURE(0.01),#9778,
'DISTANCE_ACCURACY_VALUE',
'Maximum model space distance between geometric entities at asserted c
onnectivities');
#9764=UNCERTAINTY_MEASURE_WITH_UNIT(LENGTH_MEASURE(0.01),#9778,
'DISTANCE_ACCURACY_VALUE',
'Maximum model space distance between geometric entities at asserted c
onnectivities');
#9767=(
GEOMETRIC_REPRESENTATION_CONTEXT(3)
GLOBAL_UNCERTAINTY_ASSIGNED_CONTEXT((#9754))
GLOBAL_UNIT_ASSIGNED_CONTEXT((#9778,#9780,#9781))
REPRESENTATION_CONTEXT('','3D')
);
#9777=(
GEOMETRIC_REPRESENTATION_CONTEXT(3)
GLOBAL_UNCERTAINTY_ASSIGNED_CONTEXT((#9764))
GLOBAL_UNIT_ASSIGNED_CONTEXT((#9778,#9780,#9781))
REPRESENTATION_CONTEXT('','3D')
);
#9778=(
LENGTH_UNIT()
NAMED_UNIT(*)
SI_UNIT(.MILLI.,.METRE.)
);
#9780=(
NAMED_UNIT(*)
PLANE_ANGLE_UNIT()
SI_UNIT($,.RADIAN.)
);
#9781=(
NAMED_UNIT(*)
SI_UNIT($,.STERADIAN.)
SOLID_ANGLE_UNIT()
);
#9784=SHAPE_DEFINITION_REPRESENTATION(#9796,#9858);
#9796=PRODUCT_DEFINITION_SHAPE('',$,#9871);
#9858=SHAPE_REPRESENTATION('',(#4009),#9767);
#9868=PRODUCT_DEFINITION_CONTEXT('part definition',#9906,'design');
#9871=PRODUCT_DEFINITION('Frame rail','Frame rail',#9883,#9868);
#9883=PRODUCT_DEFINITION_FORMATION('',$,#9910);
#9906=APPLICATION_CONTEXT(
'Core Data for Automotive Mechanical Design Process');
#9907=PRODUCT_CONTEXT('part definition',#9906,'mechanical');
#9910=PRODUCT('Frame rail','Frame rail',
'Independent aluminum extrusion section. Whole-mm nominal die dimensio
ns; parametric saw-cut length. Select structural loading, tolerances a
nd finish for the assembly application.',(#9907));
#9922=PRESENTATION_STYLE_ASSIGNMENT((#9933));
#9933=SURFACE_STYLE_USAGE(.BOTH.,#9944);
#9944=SURFACE_SIDE_STYLE('',(#9955));
#9955=SURFACE_STYLE_FILL_AREA(#9966);
#9966=FILL_AREA_STYLE('Dark blue',(#9977));
#9977=FILL_AREA_STYLE_COLOUR('Dark blue',#9988);
#9988=COLOUR_RGB('Dark blue',0.0901960784313725,0.270588235294118,0.513725490196078);
ENDSEC;
END-ISO-10303-21;
